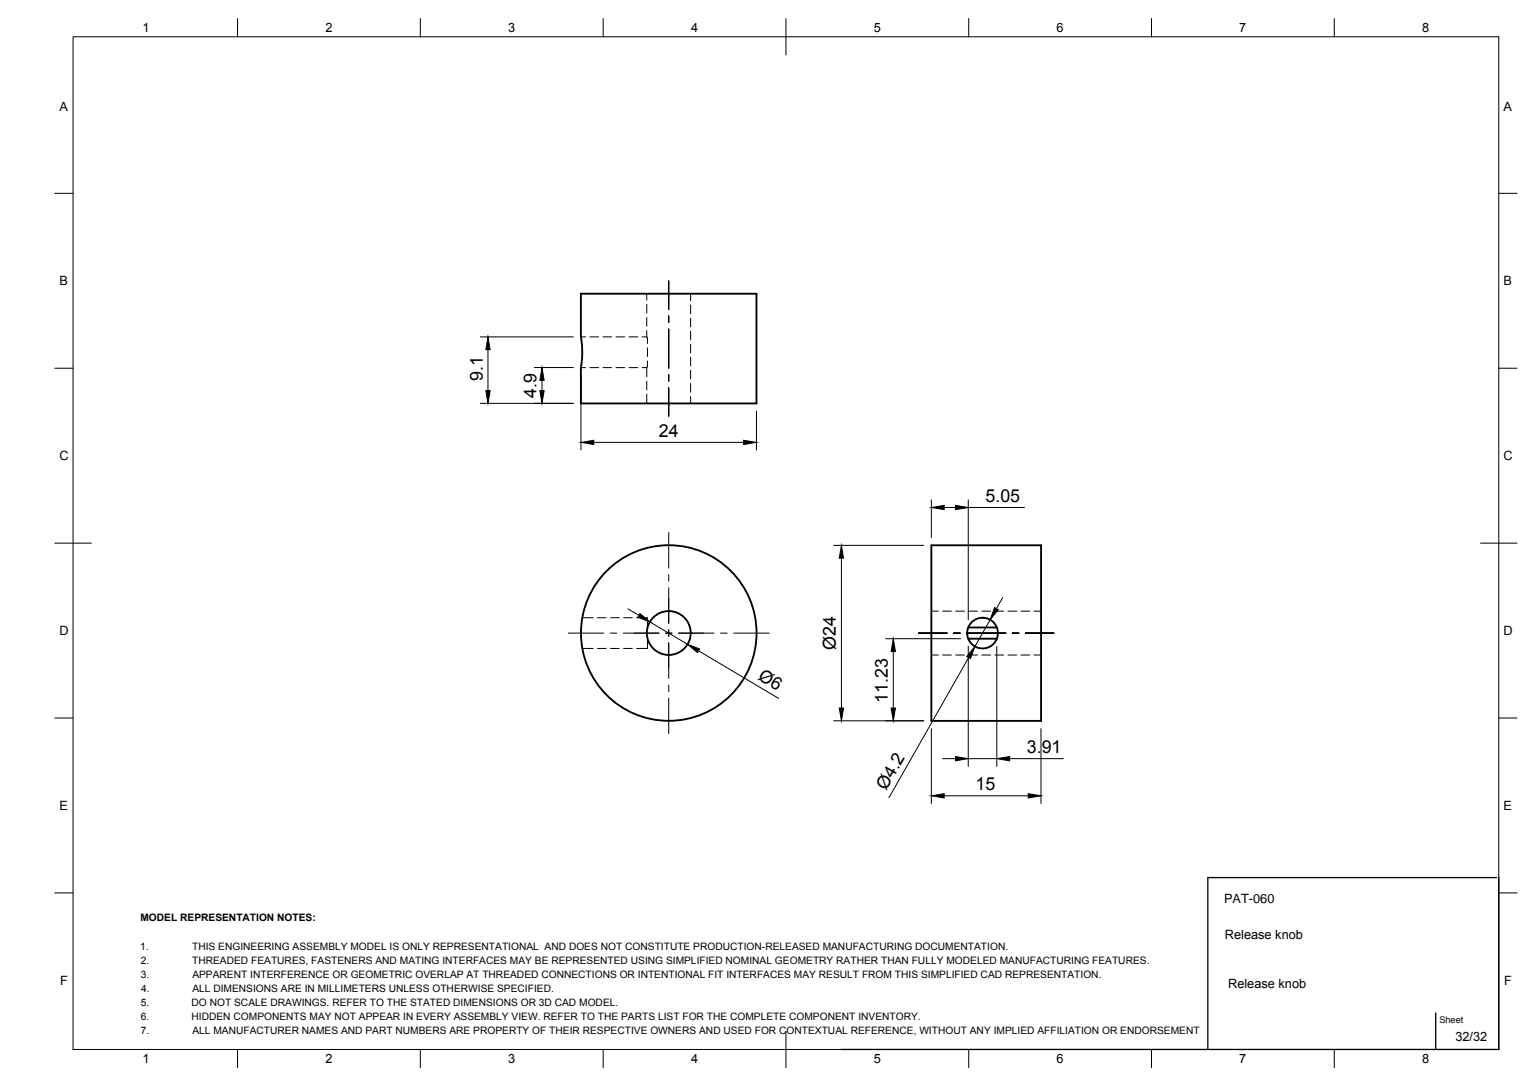
ISO-10303-21;
HEADER;
/* Generated by software containing ST-Developer
 * from STEP Tools, Inc. (www.steptools.com) 
 */

FILE_DESCRIPTION(
/* description */ ('Indexing fixture plate with plunger'),
/* implementation_level */ '2;1');

FILE_NAME(
/* name */ 'Release knob.step',
/* time_stamp */ '2026-10-28T03:23:41-07:00',
/* author */ (''),
/* organization */ (''),
/* preprocessor_version */ 'ST-DEVELOPER v20.2',
/* originating_system */ 'Autodesk Translation Framework v15.17.0.0',
/* authorisation */ '');

FILE_SCHEMA (('AUTOMOTIVE_DESIGN { 1 0 10303 214 3 1 1 }'));
ENDSEC;

DATA;
#10=MECHANICAL_DESIGN_GEOMETRIC_PRESENTATION_REPRESENTATION('',(#351),#10020);
#258=B_SPLINE_CURVE_WITH_KNOTS('',3,(#9823,#9824,#9825,#9826,#9827,#9828),
 .UNSPECIFIED.,.F.,.F.,(4,2,4),(0.917424161667463,0.994436039000116,1.07144791633277),
 .UNSPECIFIED.);
#259=B_SPLINE_CURVE_WITH_KNOTS('',3,(#9832,#9833,#9834,#9835),
 .UNSPECIFIED.,.F.,.F.,(4,4),(0.331478679666705,0.408490556999359),
 .UNSPECIFIED.);
#260=B_SPLINE_CURVE_WITH_KNOTS('',3,(#9839,#9840,#9841,#9842,#9843,#9844,
#9845,#9846,#9847,#9848,#9849,#9850,#9851,#9852,#9853,#9854,#9855,#9856,
#9857,#9858,#9859,#9860,#9861,#9862,#9863,#9864),.UNSPECIFIED.,.F.,.F.,
(4,2,2,2,2,2,2,2,2,2,2,2,4),(0.,0.0792812130427881,0.158562426085576,0.237841058284634,
0.317119690483691,0.396398322682749,0.475676954881806,0.554958167924595,
0.634239380967383,0.713520594010171,0.792801807052959,0.872080439252016,
0.951359071451074),.UNSPECIFIED.);
#261=B_SPLINE_CURVE_WITH_KNOTS('',3,(#9865,#9866,#9867,#9868,#9869,#9870,
#9871,#9872,#9873,#9874),.UNSPECIFIED.,.F.,.F.,(4,2,2,2,4),(0.951359071451074,
1.03063770365013,1.10991633584919,1.18919754889198,1.26847876193477),
 .UNSPECIFIED.);
#262=B_SPLINE_CURVE_WITH_KNOTS('',3,(#9875,#9876,#9877,#9878),
 .UNSPECIFIED.,.F.,.F.,(4,4),(0.254466802334052,0.331478679666705),
 .UNSPECIFIED.);
#288=SHAPE_REPRESENTATION_RELATIONSHIP('SRR','None',#10165,#315);
#315=ADVANCED_BREP_SHAPE_REPRESENTATION('',(#385),#10018);
#351=STYLED_ITEM('',(#10354),#385);
#385=MANIFOLD_SOLID_BREP('Body1',#4607);
#532=FACE_BOUND('',#1372,.T.);
#533=FACE_BOUND('',#1374,.T.);
#534=FACE_BOUND('',#1376,.T.);
#535=FACE_BOUND('',#1378,.T.);
#657=PLANE('',#5537);
#658=PLANE('',#5541);
#659=PLANE('',#5548);
#660=PLANE('',#5549);
#937=FACE_OUTER_BOUND('',#1368,.T.);
#938=FACE_OUTER_BOUND('',#1369,.T.);
#939=FACE_OUTER_BOUND('',#1370,.T.);
#940=FACE_OUTER_BOUND('',#1371,.T.);
#941=FACE_OUTER_BOUND('',#1373,.T.);
#942=FACE_OUTER_BOUND('',#1375,.T.);
#943=FACE_OUTER_BOUND('',#1377,.T.);
#1368=EDGE_LOOP('',(#4085,#4086));
#1369=EDGE_LOOP('',(#4087,#4088,#4089,#4090,#4091,#4092,#4093,#4094,#4095));
#1370=EDGE_LOOP('',(#4096,#4097));
#1371=EDGE_LOOP('',(#4098,#4099,#4100,#4101));
#1372=EDGE_LOOP('',(#4102,#4103,#4104,#4105,#4106));
#1373=EDGE_LOOP('',(#4107,#4108,#4109,#4110));
#1374=EDGE_LOOP('',(#4111,#4112));
#1375=EDGE_LOOP('',(#4113));
#1376=EDGE_LOOP('',(#4114));
#1377=EDGE_LOOP('',(#4115));
#1378=EDGE_LOOP('',(#4116));
#1586=LINE('',#9819,#1806);
#1587=LINE('',#9837,#1807);
#1588=LINE('',#9880,#1808);
#1589=LINE('',#9885,#1809);
#1590=LINE('',#9891,#1810);
#1806=VECTOR('',#7029,1.);
#1807=VECTOR('',#7036,0.21);
#1808=VECTOR('',#7039,1.);
#1809=VECTOR('',#7044,0.3);
#1810=VECTOR('',#7051,1.2);
#2125=CIRCLE('',#5538,0.21);
#2126=CIRCLE('',#5540,0.21);
#2127=CIRCLE('',#5543,0.3);
#2128=CIRCLE('',#5544,0.3);
#2129=CIRCLE('',#5546,1.2);
#2130=CIRCLE('',#5547,1.2);
#2484=VERTEX_POINT('',#9817);
#2485=VERTEX_POINT('',#9818);
#2486=VERTEX_POINT('',#9822);
#2487=VERTEX_POINT('',#9829);
#2488=VERTEX_POINT('',#9831);
#2489=VERTEX_POINT('',#9836);
#2490=VERTEX_POINT('',#9838);
#2491=VERTEX_POINT('',#9882);
#2492=VERTEX_POINT('',#9884);
#2493=VERTEX_POINT('',#9888);
#2494=VERTEX_POINT('',#9890);
#3022=EDGE_CURVE('',#2484,#2485,#1586,.T.);
#3023=EDGE_CURVE('',#2484,#2485,#2125,.T.);
#3024=EDGE_CURVE('',#2486,#2484,#258,.T.);
#3025=EDGE_CURVE('',#2487,#2486,#2126,.T.);
#3026=EDGE_CURVE('',#2488,#2487,#259,.T.);
#3027=EDGE_CURVE('',#2488,#2489,#1587,.T.);
#3028=EDGE_CURVE('',#2490,#2489,#260,.T.);
#3029=EDGE_CURVE('',#2489,#2490,#261,.T.);
#3030=EDGE_CURVE('',#2485,#2488,#262,.T.);
#3031=EDGE_CURVE('',#2487,#2486,#1588,.T.);
#3032=EDGE_CURVE('',#2491,#2491,#2127,.T.);
#3033=EDGE_CURVE('',#2491,#2492,#1589,.T.);
#3034=EDGE_CURVE('',#2492,#2492,#2128,.T.);
#3035=EDGE_CURVE('',#2493,#2493,#2129,.T.);
#3036=EDGE_CURVE('',#2493,#2494,#1590,.T.);
#3037=EDGE_CURVE('',#2494,#2494,#2130,.T.);
#4085=ORIENTED_EDGE('',*,*,#3022,.F.);
#4086=ORIENTED_EDGE('',*,*,#3023,.T.);
#4087=ORIENTED_EDGE('',*,*,#3024,.F.);
#4088=ORIENTED_EDGE('',*,*,#3025,.F.);
#4089=ORIENTED_EDGE('',*,*,#3026,.F.);
#4090=ORIENTED_EDGE('',*,*,#3027,.T.);
#4091=ORIENTED_EDGE('',*,*,#3028,.F.);
#4092=ORIENTED_EDGE('',*,*,#3029,.F.);
#4093=ORIENTED_EDGE('',*,*,#3027,.F.);
#4094=ORIENTED_EDGE('',*,*,#3030,.F.);
#4095=ORIENTED_EDGE('',*,*,#3023,.F.);
#4096=ORIENTED_EDGE('',*,*,#3031,.F.);
#4097=ORIENTED_EDGE('',*,*,#3025,.T.);
#4098=ORIENTED_EDGE('',*,*,#3032,.F.);
#4099=ORIENTED_EDGE('',*,*,#3033,.T.);
#4100=ORIENTED_EDGE('',*,*,#3034,.T.);
#4101=ORIENTED_EDGE('',*,*,#3033,.F.);
#4102=ORIENTED_EDGE('',*,*,#3030,.T.);
#4103=ORIENTED_EDGE('',*,*,#3026,.T.);
#4104=ORIENTED_EDGE('',*,*,#3031,.T.);
#4105=ORIENTED_EDGE('',*,*,#3024,.T.);
#4106=ORIENTED_EDGE('',*,*,#3022,.T.);
#4107=ORIENTED_EDGE('',*,*,#3035,.F.);
#4108=ORIENTED_EDGE('',*,*,#3036,.T.);
#4109=ORIENTED_EDGE('',*,*,#3037,.T.);
#4110=ORIENTED_EDGE('',*,*,#3036,.F.);
#4111=ORIENTED_EDGE('',*,*,#3028,.T.);
#4112=ORIENTED_EDGE('',*,*,#3029,.T.);
#4113=ORIENTED_EDGE('',*,*,#3035,.T.);
#4114=ORIENTED_EDGE('',*,*,#3032,.T.);
#4115=ORIENTED_EDGE('',*,*,#3037,.F.);
#4116=ORIENTED_EDGE('',*,*,#3034,.F.);
#4281=CYLINDRICAL_SURFACE('',#5539,0.21);
#4282=CYLINDRICAL_SURFACE('',#5542,0.3);
#4283=CYLINDRICAL_SURFACE('',#5545,1.2);
#4552=ADVANCED_FACE('',(#937),#657,.T.);
#4553=ADVANCED_FACE('',(#938),#4281,.F.);
#4554=ADVANCED_FACE('',(#939),#658,.T.);
#4555=ADVANCED_FACE('',(#940,#532),#4282,.F.);
#4556=ADVANCED_FACE('',(#941,#533),#4283,.T.);
#4557=ADVANCED_FACE('',(#942,#534),#659,.T.);
#4558=ADVANCED_FACE('',(#943,#535),#660,.F.);
#4607=CLOSED_SHELL('',(#4552,#4553,#4554,#4555,#4556,#4557,#4558));
#5536=AXIS2_PLACEMENT_3D('',#9815,#7025,#7026);
#5537=AXIS2_PLACEMENT_3D('',#9816,#7027,#7028);
#5538=AXIS2_PLACEMENT_3D('',#9820,#7030,#7031);
#5539=AXIS2_PLACEMENT_3D('',#9821,#7032,#7033);
#5540=AXIS2_PLACEMENT_3D('',#9830,#7034,#7035);
#5541=AXIS2_PLACEMENT_3D('',#9879,#7037,#7038);
#5542=AXIS2_PLACEMENT_3D('',#9881,#7040,#7041);
#5543=AXIS2_PLACEMENT_3D('',#9883,#7042,#7043);
#5544=AXIS2_PLACEMENT_3D('',#9886,#7045,#7046);
#5545=AXIS2_PLACEMENT_3D('',#9887,#7047,#7048);
#5546=AXIS2_PLACEMENT_3D('',#9889,#7049,#7050);
#5547=AXIS2_PLACEMENT_3D('',#9892,#7052,#7053);
#5548=AXIS2_PLACEMENT_3D('',#9893,#7054,#7055);
#5549=AXIS2_PLACEMENT_3D('',#9894,#7056,#7057);
#7025=DIRECTION('axis',(0.,0.,1.));
#7026=DIRECTION('refdir',(1.,0.,0.));
#7027=DIRECTION('center_axis',(1.,0.,0.));
#7028=DIRECTION('ref_axis',(0.,0.,-1.));
#7029=DIRECTION('',(0.,0.,1.));
#7030=DIRECTION('center_axis',(1.,0.,0.));
#7031=DIRECTION('ref_axis',(0.,0.,-1.));
#7032=DIRECTION('center_axis',(1.,0.,0.));
#7033=DIRECTION('ref_axis',(0.,0.,-1.));
#7034=DIRECTION('center_axis',(1.,0.,0.));
#7035=DIRECTION('ref_axis',(0.,0.,-1.));
#7036=DIRECTION('',(1.,0.,0.));
#7037=DIRECTION('center_axis',(1.,0.,0.));
#7038=DIRECTION('ref_axis',(0.,0.,-1.));
#7039=DIRECTION('',(0.,0.,-1.));
#7040=DIRECTION('center_axis',(0.,0.,1.));
#7041=DIRECTION('ref_axis',(1.,0.,0.));
#7042=DIRECTION('center_axis',(0.,0.,-1.));
#7043=DIRECTION('ref_axis',(1.,0.,0.));
#7044=DIRECTION('',(0.,0.,-1.));
#7045=DIRECTION('center_axis',(0.,0.,-1.));
#7046=DIRECTION('ref_axis',(1.,0.,0.));
#7047=DIRECTION('center_axis',(0.,0.,1.));
#7048=DIRECTION('ref_axis',(1.,0.,0.));
#7049=DIRECTION('center_axis',(0.,0.,1.));
#7050=DIRECTION('ref_axis',(1.,0.,0.));
#7051=DIRECTION('',(0.,0.,-1.));
#7052=DIRECTION('center_axis',(0.,0.,1.));
#7053=DIRECTION('ref_axis',(1.,0.,0.));
#7054=DIRECTION('center_axis',(0.,0.,1.));
#7055=DIRECTION('ref_axis',(1.,0.,0.));
#7056=DIRECTION('center_axis',(0.,0.,1.));
#7057=DIRECTION('ref_axis',(1.,0.,0.));
#9815=CARTESIAN_POINT('',(0.,0.,0.));
#9816=CARTESIAN_POINT('Origin',(7.49,0.,-2.2));
#9817=CARTESIAN_POINT('',(7.49,0.0768114574786819,-2.39544820285692));
#9818=CARTESIAN_POINT('',(7.49,0.0768114574786819,-2.00455179714308));
#9819=CARTESIAN_POINT('',(7.49,0.0768114574786819,-3.));
#9820=CARTESIAN_POINT('Origin',(7.49,0.,-2.2));
#9821=CARTESIAN_POINT('Origin',(7.49,0.,-2.2));
#9822=CARTESIAN_POINT('',(7.49,-0.0768114574786819,-2.39544820285692));
#9823=CARTESIAN_POINT('Ctrl Pts',(7.49,-0.0768114574786819,-2.39544820285692));
#9824=CARTESIAN_POINT('Ctrl Pts',(7.49646752117291,-0.0523934708695169,
-2.40504451079288));
#9825=CARTESIAN_POINT('Ctrl Pts',(7.5,-0.025670625777551,-2.41));
#9826=CARTESIAN_POINT('Ctrl Pts',(7.5,0.025670625777551,-2.41));
#9827=CARTESIAN_POINT('Ctrl Pts',(7.49646752117291,0.0523934708695169,-2.40504451079288));
#9828=CARTESIAN_POINT('Ctrl Pts',(7.49,0.0768114574786818,-2.39544820285692));
#9829=CARTESIAN_POINT('',(7.49,-0.0768114574786819,-2.00455179714308));
#9830=CARTESIAN_POINT('Origin',(7.49,0.,-2.2));
#9831=CARTESIAN_POINT('',(7.5,-1.63282383430008E-17,-1.99));
#9832=CARTESIAN_POINT('Ctrl Pts',(7.5,-3.46944695195361E-18,-1.99));
#9833=CARTESIAN_POINT('Ctrl Pts',(7.5,-0.0256706257775511,-1.99));
#9834=CARTESIAN_POINT('Ctrl Pts',(7.49646752117291,-0.0523934708695168,
-1.99495548920712));
#9835=CARTESIAN_POINT('Ctrl Pts',(7.49,-0.0768114574786816,-2.00455179714308));
#9836=CARTESIAN_POINT('',(8.4,-2.57175827820944E-17,-1.99));
#9837=CARTESIAN_POINT('',(7.49,-2.57175827820944E-17,-1.99));
#9838=CARTESIAN_POINT('',(8.38148212005091,0.21,-2.2));
#9839=CARTESIAN_POINT('Ctrl Pts',(8.38148212005091,0.21,-2.2));
#9840=CARTESIAN_POINT('Ctrl Pts',(8.38148212005091,0.21,-2.22642707101426));
#9841=CARTESIAN_POINT('Ctrl Pts',(8.38246056146673,0.204707379175836,-2.25457755408867));
#9842=CARTESIAN_POINT('Ctrl Pts',(8.38597389417424,0.183259409780014,-2.30630056955556));
#9843=CARTESIAN_POINT('Ctrl Pts',(8.38845578531258,0.167106958412512,-2.32987788968584));
#9844=CARTESIAN_POINT('Ctrl Pts',(8.3930982535617,0.129878495645339,-2.36710635245301));
#9845=CARTESIAN_POINT('Ctrl Pts',(8.39556345497295,0.106300916040875,-2.38325927901602));
#9846=CARTESIAN_POINT('Ctrl Pts',(8.39903845223025,0.0545770066794469,-2.40470759325685));
#9847=CARTESIAN_POINT('Ctrl Pts',(8.4,0.0264262107330192,-2.41));
#9848=CARTESIAN_POINT('Ctrl Pts',(8.4,-0.0264262107330192,-2.41));
#9849=CARTESIAN_POINT('Ctrl Pts',(8.39903845223025,-0.0545770066794469,
-2.40470759325685));
#9850=CARTESIAN_POINT('Ctrl Pts',(8.39556345497295,-0.106300916040875,-2.38325927901602));
#9851=CARTESIAN_POINT('Ctrl Pts',(8.3930982535617,-0.129878495645339,-2.36710635245301));
#9852=CARTESIAN_POINT('Ctrl Pts',(8.38845578531258,-0.167106958412512,-2.32987788968584));
#9853=CARTESIAN_POINT('Ctrl Pts',(8.38597389417424,-0.183259409780014,-2.30630056955556));
#9854=CARTESIAN_POINT('Ctrl Pts',(8.38246056146673,-0.204707379175836,-2.25457755408867));
#9855=CARTESIAN_POINT('Ctrl Pts',(8.38148212005091,-0.21,-2.22642707101426));
#9856=CARTESIAN_POINT('Ctrl Pts',(8.38148212005091,-0.21,-2.17357292898574));
#9857=CARTESIAN_POINT('Ctrl Pts',(8.38246056146673,-0.204707379175836,-2.14542244591133));
#9858=CARTESIAN_POINT('Ctrl Pts',(8.38597389417424,-0.183259409780014,-2.09369943044444));
#9859=CARTESIAN_POINT('Ctrl Pts',(8.38845578531258,-0.167106958412512,-2.07012211031416));
#9860=CARTESIAN_POINT('Ctrl Pts',(8.3930982535617,-0.129878495645339,-2.03289364754699));
#9861=CARTESIAN_POINT('Ctrl Pts',(8.39556345497295,-0.106300916040875,-2.01674072098398));
#9862=CARTESIAN_POINT('Ctrl Pts',(8.39903845223025,-0.0545770066794469,
-1.99529240674315));
#9863=CARTESIAN_POINT('Ctrl Pts',(8.4,-0.0264262107330192,-1.99));
#9864=CARTESIAN_POINT('Ctrl Pts',(8.4,-4.85722573273506E-17,-1.99));
#9865=CARTESIAN_POINT('Ctrl Pts',(8.4,-8.32667268468867E-17,-1.99));
#9866=CARTESIAN_POINT('Ctrl Pts',(8.4,0.0264262107330192,-1.99));
#9867=CARTESIAN_POINT('Ctrl Pts',(8.39903845223025,0.0545770066794466,-1.99529240674315));
#9868=CARTESIAN_POINT('Ctrl Pts',(8.39556345497295,0.106300916040875,-2.01674072098398));
#9869=CARTESIAN_POINT('Ctrl Pts',(8.3930982535617,0.129878495645339,-2.03289364754699));
#9870=CARTESIAN_POINT('Ctrl Pts',(8.38845578531258,0.167106958412512,-2.07012211031416));
#9871=CARTESIAN_POINT('Ctrl Pts',(8.38597389417424,0.183259409780014,-2.09369943044444));
#9872=CARTESIAN_POINT('Ctrl Pts',(8.38246056146673,0.204707379175836,-2.14542244591133));
#9873=CARTESIAN_POINT('Ctrl Pts',(8.38148212005091,0.21,-2.17357292898574));
#9874=CARTESIAN_POINT('Ctrl Pts',(8.38148212005091,0.21,-2.2));
#9875=CARTESIAN_POINT('Ctrl Pts',(7.49,0.0768114574786816,-2.00455179714308));
#9876=CARTESIAN_POINT('Ctrl Pts',(7.49646752117291,0.0523934708695167,-1.99495548920712));
#9877=CARTESIAN_POINT('Ctrl Pts',(7.5,0.025670625777551,-1.99));
#9878=CARTESIAN_POINT('Ctrl Pts',(7.5,-5.55111512312578E-17,-1.99));
#9879=CARTESIAN_POINT('Origin',(7.49,0.,-2.2));
#9880=CARTESIAN_POINT('',(7.49,-0.0768114574786819,-3.));
#9881=CARTESIAN_POINT('Origin',(7.2,0.,-3.));
#9882=CARTESIAN_POINT('',(6.9,-3.67394039744206E-17,-1.5));
#9883=CARTESIAN_POINT('Origin',(7.2,0.,-1.5));
#9884=CARTESIAN_POINT('',(6.9,-3.67394039744206E-17,-3.));
#9885=CARTESIAN_POINT('',(6.9,-3.67394039744206E-17,-3.));
#9886=CARTESIAN_POINT('Origin',(7.2,0.,-3.));
#9887=CARTESIAN_POINT('Origin',(7.2,0.,-3.));
#9888=CARTESIAN_POINT('',(6.,-1.46957615897682E-16,-1.5));
#9889=CARTESIAN_POINT('Origin',(7.2,0.,-1.5));
#9890=CARTESIAN_POINT('',(6.,-1.46957615897682E-16,-3.));
#9891=CARTESIAN_POINT('',(6.,-1.46957615897682E-16,-3.));
#9892=CARTESIAN_POINT('Origin',(7.2,0.,-3.));
#9893=CARTESIAN_POINT('Origin',(7.2,0.,-1.5));
#9894=CARTESIAN_POINT('Origin',(7.2,0.,-3.));
#9985=UNCERTAINTY_MEASURE_WITH_UNIT(LENGTH_MEASURE(0.001),#10021,
'DISTANCE_ACCURACY_VALUE',
'Maximum model space distance between geometric entities at asserted c
onnectivities');
#9987=UNCERTAINTY_MEASURE_WITH_UNIT(LENGTH_MEASURE(0.001),#10021,
'DISTANCE_ACCURACY_VALUE',
'Maximum model space distance between geometric entities at asserted c
onnectivities');
#10018=(
GEOMETRIC_REPRESENTATION_CONTEXT(3)
GLOBAL_UNCERTAINTY_ASSIGNED_CONTEXT((#9985))
GLOBAL_UNIT_ASSIGNED_CONTEXT((#10021,#10023,#10024))
REPRESENTATION_CONTEXT('','3D')
);
#10020=(
GEOMETRIC_REPRESENTATION_CONTEXT(3)
GLOBAL_UNCERTAINTY_ASSIGNED_CONTEXT((#9987))
GLOBAL_UNIT_ASSIGNED_CONTEXT((#10021,#10023,#10024))
REPRESENTATION_CONTEXT('','3D')
);
#10021=(
LENGTH_UNIT()
NAMED_UNIT(*)
SI_UNIT(.CENTI.,.METRE.)
);
#10023=(
NAMED_UNIT(*)
PLANE_ANGLE_UNIT()
SI_UNIT($,.RADIAN.)
);
#10024=(
NAMED_UNIT(*)
SI_UNIT($,.STERADIAN.)
SOLID_ANGLE_UNIT()
);
#10055=SHAPE_DEFINITION_REPRESENTATION(#10127,#10165);
#10127=PRODUCT_DEFINITION_SHAPE('',$,#10198);
#10165=SHAPE_REPRESENTATION('',(#5536),#10018);
#10167=PRODUCT_DEFINITION_CONTEXT('part definition',#10265,'design');
#10198=PRODUCT_DEFINITION('Release knob','Release knob',#10230,#10167);
#10230=PRODUCT_DEFINITION_FORMATION('',$,#10297);
#10265=APPLICATION_CONTEXT(
'Core Data for Automotive Mechanical Design Process');
#10266=PRODUCT_CONTEXT('part definition',#10265,'mechanical');
#10297=PRODUCT('Release knob','Release knob','Release knob',(#10266));
#10348=COLOUR_RGB('Light Blue',0.38,0.62,0.78);
#10349=FILL_AREA_STYLE_COLOUR('',#10348);
#10350=FILL_AREA_STYLE('',(#10349));
#10351=SURFACE_STYLE_FILL_AREA(#10350);
#10352=SURFACE_SIDE_STYLE('',(#10351));
#10353=SURFACE_STYLE_USAGE(.BOTH.,#10352);
#10354=PRESENTATION_STYLE_ASSIGNMENT((#10353));
ENDSEC;
END-ISO-10303-21;
